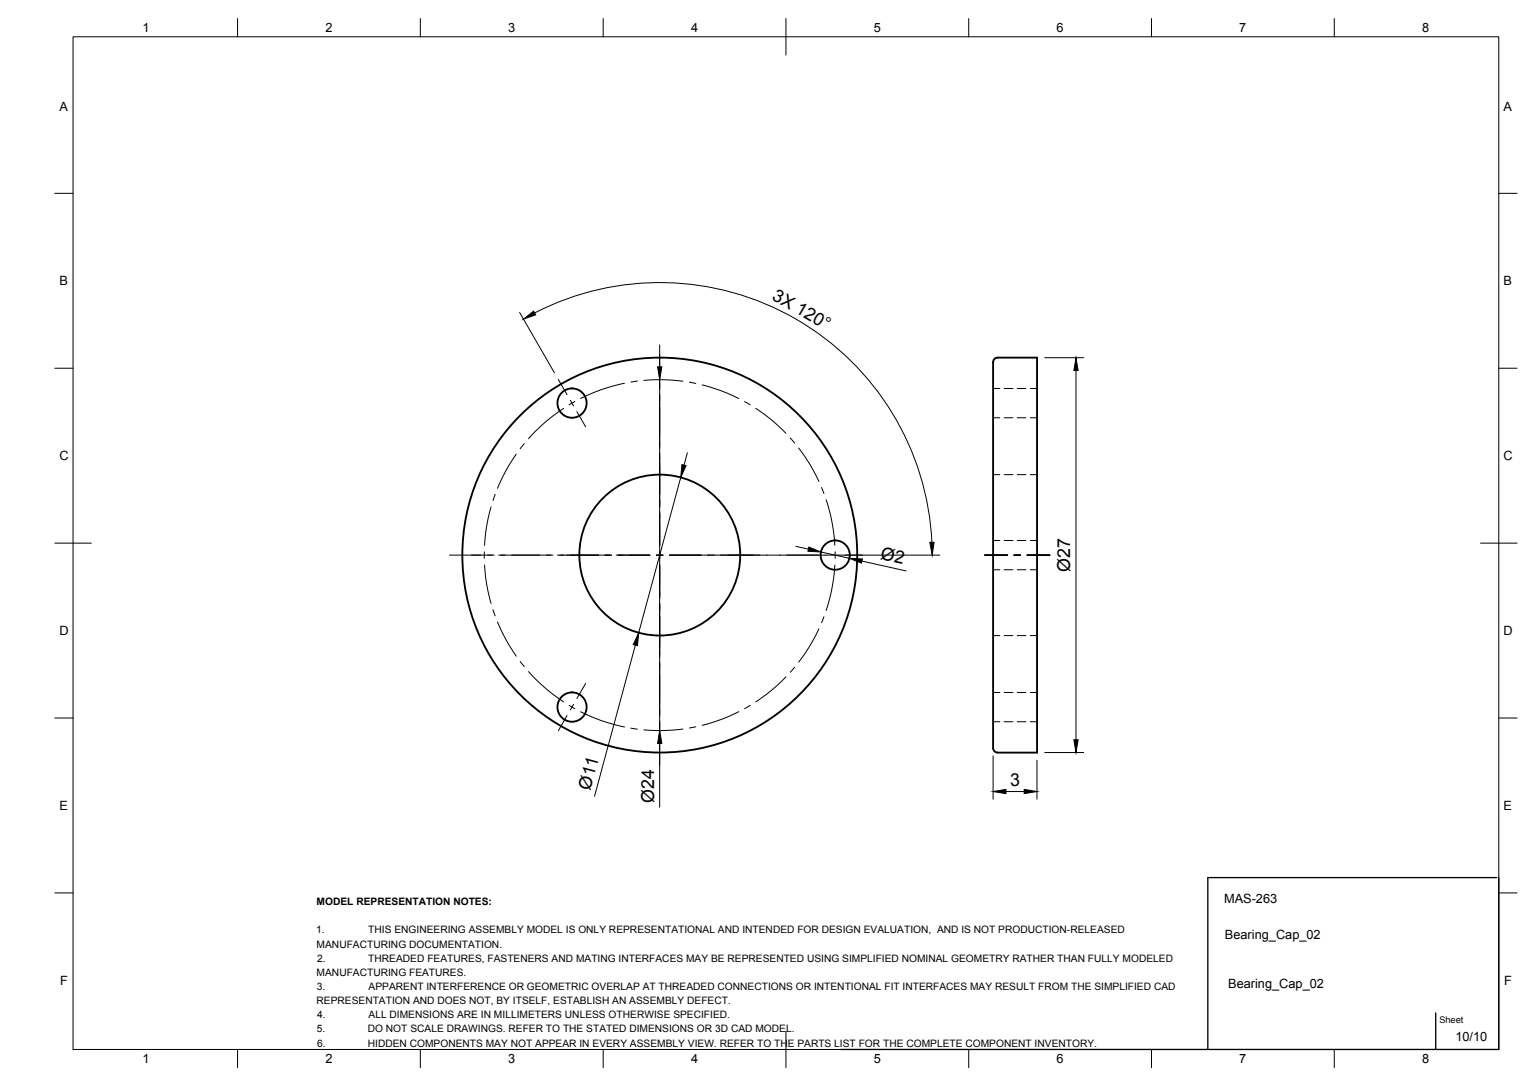
ISO-10303-21;
HEADER;
/* Generated by software containing ST-Developer
 * from STEP Tools, Inc. (www.steptools.com) 
 */

FILE_DESCRIPTION(
/* description */ (''),
/* implementation_level */ '2;1');

FILE_NAME(
/* name */ 'Bearing_Cap_02.step',
/* time_stamp */ '2026-10-12T15:47:30-07:00',
/* author */ (''),
/* organization */ (''),
/* preprocessor_version */ 'ST-DEVELOPER v20.2',
/* originating_system */ 'Autodesk Translation Framework v15.15.0.0',
/* authorisation */ '');

FILE_SCHEMA (('AUTOMOTIVE_DESIGN { 1 0 10303 214 3 1 1 }'));
ENDSEC;

DATA;
#10=MECHANICAL_DESIGN_GEOMETRIC_PRESENTATION_REPRESENTATION('',(#88),#88483);
#70=SHAPE_REPRESENTATION_RELATIONSHIP('SRR','None',#88526,#79);
#79=ADVANCED_BREP_SHAPE_REPRESENTATION('',(#123),#88480);
#88=STYLED_ITEM('',(#88574),#123);
#123=MANIFOLD_SOLID_BREP('Body1',#12998);
#174=TOROIDAL_SURFACE('',#13981,13.2,0.3);
#399=FACE_BOUND('',#2026,.T.);
#400=FACE_BOUND('',#2027,.T.);
#401=FACE_BOUND('',#2028,.T.);
#402=FACE_BOUND('',#2029,.T.);
#403=FACE_BOUND('',#2032,.T.);
#404=FACE_BOUND('',#2033,.T.);
#405=FACE_BOUND('',#2034,.T.);
#406=FACE_BOUND('',#2035,.T.);
#551=PLANE('',#13988);
#552=PLANE('',#13992);
#1302=FACE_OUTER_BOUND('',#2020,.T.);
#1303=FACE_OUTER_BOUND('',#2021,.T.);
#1304=FACE_OUTER_BOUND('',#2022,.T.);
#1305=FACE_OUTER_BOUND('',#2023,.T.);
#1306=FACE_OUTER_BOUND('',#2024,.T.);
#1307=FACE_OUTER_BOUND('',#2025,.T.);
#1308=FACE_OUTER_BOUND('',#2030,.T.);
#1309=FACE_OUTER_BOUND('',#2031,.T.);
#2020=EDGE_LOOP('',(#11452,#11453,#11454,#11455));
#2021=EDGE_LOOP('',(#11456,#11457,#11458,#11459));
#2022=EDGE_LOOP('',(#11460,#11461,#11462,#11463));
#2023=EDGE_LOOP('',(#11464,#11465,#11466,#11467,#11468));
#2024=EDGE_LOOP('',(#11469,#11470,#11471,#11472,#11473));
#2025=EDGE_LOOP('',(#11474));
#2026=EDGE_LOOP('',(#11475));
#2027=EDGE_LOOP('',(#11476));
#2028=EDGE_LOOP('',(#11477));
#2029=EDGE_LOOP('',(#11478));
#2030=EDGE_LOOP('',(#11479,#11480,#11481,#11482));
#2031=EDGE_LOOP('',(#11483));
#2032=EDGE_LOOP('',(#11484));
#2033=EDGE_LOOP('',(#11485));
#2034=EDGE_LOOP('',(#11486));
#2035=EDGE_LOOP('',(#11487));
#2686=CIRCLE('',#13973,1.);
#2687=CIRCLE('',#13974,1.);
#2688=CIRCLE('',#13976,1.);
#2689=CIRCLE('',#13977,1.);
#2690=CIRCLE('',#13979,1.);
#2691=CIRCLE('',#13980,1.);
#2692=CIRCLE('',#13982,13.2);
#2693=CIRCLE('',#13983,0.3);
#2694=CIRCLE('',#13984,13.5);
#2695=CIRCLE('',#13985,13.5);
#2696=CIRCLE('',#13987,13.5);
#2697=CIRCLE('',#13989,5.5);
#2698=CIRCLE('',#13991,5.5);
#4089=LINE('',#87468,#4559);
#4090=LINE('',#87474,#4560);
#4091=LINE('',#87480,#4561);
#4092=LINE('',#87493,#4562);
#4093=LINE('',#87499,#4563);
#4559=VECTOR('',#16487,1.);
#4560=VECTOR('',#16494,1.);
#4561=VECTOR('',#16501,1.);
#4562=VECTOR('',#16518,13.5);
#4563=VECTOR('',#16525,5.5);
#5821=VERTEX_POINT('',#87465);
#5822=VERTEX_POINT('',#87467);
#5823=VERTEX_POINT('',#87471);
#5824=VERTEX_POINT('',#87473);
#5825=VERTEX_POINT('',#87477);
#5826=VERTEX_POINT('',#87479);
#5827=VERTEX_POINT('',#87483);
#5828=VERTEX_POINT('',#87485);
#5829=VERTEX_POINT('',#87487);
#5830=VERTEX_POINT('',#87491);
#5831=VERTEX_POINT('',#87495);
#5832=VERTEX_POINT('',#87498);
#7738=EDGE_CURVE('',#5821,#5821,#2686,.T.);
#7739=EDGE_CURVE('',#5821,#5822,#4089,.T.);
#7740=EDGE_CURVE('',#5822,#5822,#2687,.T.);
#7741=EDGE_CURVE('',#5823,#5823,#2688,.T.);
#7742=EDGE_CURVE('',#5823,#5824,#4090,.T.);
#7743=EDGE_CURVE('',#5824,#5824,#2689,.T.);
#7744=EDGE_CURVE('',#5825,#5825,#2690,.T.);
#7745=EDGE_CURVE('',#5825,#5826,#4091,.T.);
#7746=EDGE_CURVE('',#5826,#5826,#2691,.T.);
#7747=EDGE_CURVE('',#5827,#5827,#2692,.T.);
#7748=EDGE_CURVE('',#5827,#5828,#2693,.T.);
#7749=EDGE_CURVE('',#5829,#5828,#2694,.T.);
#7750=EDGE_CURVE('',#5828,#5829,#2695,.T.);
#7751=EDGE_CURVE('',#5830,#5830,#2696,.T.);
#7752=EDGE_CURVE('',#5830,#5829,#4092,.T.);
#7753=EDGE_CURVE('',#5831,#5831,#2697,.T.);
#7754=EDGE_CURVE('',#5831,#5832,#4093,.T.);
#7755=EDGE_CURVE('',#5832,#5832,#2698,.T.);
#11452=ORIENTED_EDGE('',*,*,#7738,.T.);
#11453=ORIENTED_EDGE('',*,*,#7739,.T.);
#11454=ORIENTED_EDGE('',*,*,#7740,.T.);
#11455=ORIENTED_EDGE('',*,*,#7739,.F.);
#11456=ORIENTED_EDGE('',*,*,#7741,.T.);
#11457=ORIENTED_EDGE('',*,*,#7742,.T.);
#11458=ORIENTED_EDGE('',*,*,#7743,.T.);
#11459=ORIENTED_EDGE('',*,*,#7742,.F.);
#11460=ORIENTED_EDGE('',*,*,#7744,.T.);
#11461=ORIENTED_EDGE('',*,*,#7745,.T.);
#11462=ORIENTED_EDGE('',*,*,#7746,.T.);
#11463=ORIENTED_EDGE('',*,*,#7745,.F.);
#11464=ORIENTED_EDGE('',*,*,#7747,.F.);
#11465=ORIENTED_EDGE('',*,*,#7748,.T.);
#11466=ORIENTED_EDGE('',*,*,#7749,.F.);
#11467=ORIENTED_EDGE('',*,*,#7750,.F.);
#11468=ORIENTED_EDGE('',*,*,#7748,.F.);
#11469=ORIENTED_EDGE('',*,*,#7751,.F.);
#11470=ORIENTED_EDGE('',*,*,#7752,.T.);
#11471=ORIENTED_EDGE('',*,*,#7749,.T.);
#11472=ORIENTED_EDGE('',*,*,#7750,.T.);
#11473=ORIENTED_EDGE('',*,*,#7752,.F.);
#11474=ORIENTED_EDGE('',*,*,#7747,.T.);
#11475=ORIENTED_EDGE('',*,*,#7740,.F.);
#11476=ORIENTED_EDGE('',*,*,#7743,.F.);
#11477=ORIENTED_EDGE('',*,*,#7746,.F.);
#11478=ORIENTED_EDGE('',*,*,#7753,.F.);
#11479=ORIENTED_EDGE('',*,*,#7753,.T.);
#11480=ORIENTED_EDGE('',*,*,#7754,.T.);
#11481=ORIENTED_EDGE('',*,*,#7755,.F.);
#11482=ORIENTED_EDGE('',*,*,#7754,.F.);
#11483=ORIENTED_EDGE('',*,*,#7751,.T.);
#11484=ORIENTED_EDGE('',*,*,#7738,.F.);
#11485=ORIENTED_EDGE('',*,*,#7741,.F.);
#11486=ORIENTED_EDGE('',*,*,#7744,.F.);
#11487=ORIENTED_EDGE('',*,*,#7755,.T.);
#12271=CYLINDRICAL_SURFACE('',#13972,1.);
#12272=CYLINDRICAL_SURFACE('',#13975,1.);
#12273=CYLINDRICAL_SURFACE('',#13978,1.);
#12274=CYLINDRICAL_SURFACE('',#13986,13.5);
#12275=CYLINDRICAL_SURFACE('',#13990,5.5);
#12832=ADVANCED_FACE('',(#1302),#12271,.F.);
#12833=ADVANCED_FACE('',(#1303),#12272,.F.);
#12834=ADVANCED_FACE('',(#1304),#12273,.F.);
#12835=ADVANCED_FACE('',(#1305),#174,.T.);
#12836=ADVANCED_FACE('',(#1306),#12274,.T.);
#12837=ADVANCED_FACE('',(#1307,#399,#400,#401,#402),#551,.F.);
#12838=ADVANCED_FACE('',(#1308),#12275,.F.);
#12839=ADVANCED_FACE('',(#1309,#403,#404,#405,#406),#552,.T.);
#12998=CLOSED_SHELL('',(#12832,#12833,#12834,#12835,#12836,#12837,#12838,
#12839));
#13971=AXIS2_PLACEMENT_3D('',#87463,#16481,#16482);
#13972=AXIS2_PLACEMENT_3D('',#87464,#16483,#16484);
#13973=AXIS2_PLACEMENT_3D('',#87466,#16485,#16486);
#13974=AXIS2_PLACEMENT_3D('',#87469,#16488,#16489);
#13975=AXIS2_PLACEMENT_3D('',#87470,#16490,#16491);
#13976=AXIS2_PLACEMENT_3D('',#87472,#16492,#16493);
#13977=AXIS2_PLACEMENT_3D('',#87475,#16495,#16496);
#13978=AXIS2_PLACEMENT_3D('',#87476,#16497,#16498);
#13979=AXIS2_PLACEMENT_3D('',#87478,#16499,#16500);
#13980=AXIS2_PLACEMENT_3D('',#87481,#16502,#16503);
#13981=AXIS2_PLACEMENT_3D('',#87482,#16504,#16505);
#13982=AXIS2_PLACEMENT_3D('',#87484,#16506,#16507);
#13983=AXIS2_PLACEMENT_3D('',#87486,#16508,#16509);
#13984=AXIS2_PLACEMENT_3D('',#87488,#16510,#16511);
#13985=AXIS2_PLACEMENT_3D('',#87489,#16512,#16513);
#13986=AXIS2_PLACEMENT_3D('',#87490,#16514,#16515);
#13987=AXIS2_PLACEMENT_3D('',#87492,#16516,#16517);
#13988=AXIS2_PLACEMENT_3D('',#87494,#16519,#16520);
#13989=AXIS2_PLACEMENT_3D('',#87496,#16521,#16522);
#13990=AXIS2_PLACEMENT_3D('',#87497,#16523,#16524);
#13991=AXIS2_PLACEMENT_3D('',#87500,#16526,#16527);
#13992=AXIS2_PLACEMENT_3D('',#87501,#16528,#16529);
#16481=DIRECTION('axis',(0.,0.,1.));
#16482=DIRECTION('refdir',(1.,0.,0.));
#16483=DIRECTION('center_axis',(-1.,0.,0.));
#16484=DIRECTION('ref_axis',(0.,1.,0.));
#16485=DIRECTION('center_axis',(1.,0.,0.));
#16486=DIRECTION('ref_axis',(0.,1.,0.));
#16487=DIRECTION('',(-1.,0.,0.));
#16488=DIRECTION('center_axis',(-1.,0.,0.));
#16489=DIRECTION('ref_axis',(0.,1.,0.));
#16490=DIRECTION('center_axis',(-1.,0.,0.));
#16491=DIRECTION('ref_axis',(0.,1.,0.));
#16492=DIRECTION('center_axis',(1.,0.,0.));
#16493=DIRECTION('ref_axis',(0.,1.,0.));
#16494=DIRECTION('',(-1.,0.,0.));
#16495=DIRECTION('center_axis',(-1.,0.,0.));
#16496=DIRECTION('ref_axis',(0.,1.,0.));
#16497=DIRECTION('center_axis',(-1.,0.,0.));
#16498=DIRECTION('ref_axis',(0.,1.,0.));
#16499=DIRECTION('center_axis',(1.,0.,0.));
#16500=DIRECTION('ref_axis',(0.,1.,0.));
#16501=DIRECTION('',(-1.,0.,0.));
#16502=DIRECTION('center_axis',(-1.,0.,0.));
#16503=DIRECTION('ref_axis',(0.,1.,0.));
#16504=DIRECTION('center_axis',(-1.,0.,0.));
#16505=DIRECTION('ref_axis',(0.,0.,-1.));
#16506=DIRECTION('center_axis',(-1.,0.,0.));
#16507=DIRECTION('ref_axis',(0.,0.342020143325669,0.939692620785908));
#16508=DIRECTION('center_axis',(0.,1.,0.));
#16509=DIRECTION('ref_axis',(0.,0.,1.));
#16510=DIRECTION('center_axis',(1.,0.,0.));
#16511=DIRECTION('ref_axis',(0.,0.342020143325669,0.939692620785908));
#16512=DIRECTION('center_axis',(1.,0.,0.));
#16513=DIRECTION('ref_axis',(0.,0.342020143325669,0.939692620785908));
#16514=DIRECTION('center_axis',(1.,0.,0.));
#16515=DIRECTION('ref_axis',(0.,-0.296296296296299,-0.955096070979823));
#16516=DIRECTION('center_axis',(1.,0.,0.));
#16517=DIRECTION('ref_axis',(0.,-0.296296296296299,-0.955096070979823));
#16518=DIRECTION('',(-1.,0.,0.));
#16519=DIRECTION('center_axis',(1.,0.,0.));
#16520=DIRECTION('ref_axis',(0.,1.,0.));
#16521=DIRECTION('center_axis',(-1.,0.,0.));
#16522=DIRECTION('ref_axis',(0.,1.,0.));
#16523=DIRECTION('center_axis',(1.,0.,0.));
#16524=DIRECTION('ref_axis',(0.,1.,0.));
#16525=DIRECTION('',(1.,0.,0.));
#16526=DIRECTION('center_axis',(-1.,0.,0.));
#16527=DIRECTION('ref_axis',(0.,1.,0.));
#16528=DIRECTION('center_axis',(1.,0.,0.));
#16529=DIRECTION('ref_axis',(0.,1.,0.));
#87463=CARTESIAN_POINT('',(0.,0.,0.));
#87464=CARTESIAN_POINT('Origin',(-26.3408711739,15.6090782051017,5.99920149541289));
#87465=CARTESIAN_POINT('',(-23.3408711739,14.6090782051017,5.99920149541289));
#87466=CARTESIAN_POINT('Origin',(-23.3408711739,15.6090782051017,5.99920149541289));
#87467=CARTESIAN_POINT('',(-26.3408711739,14.6090782051017,5.99920149541289));
#87468=CARTESIAN_POINT('',(-26.3408711739,14.6090782051017,5.99920149541289));
#87469=CARTESIAN_POINT('Origin',(-26.3408711739,15.6090782051017,5.99920149541289));
#87470=CARTESIAN_POINT('Origin',(-26.3408711739,36.3909217948983,5.99920149541289));
#87471=CARTESIAN_POINT('',(-23.3408711739,35.3909217948983,5.99920149541289));
#87472=CARTESIAN_POINT('Origin',(-23.3408711739,36.3909217948983,5.99920149541289));
#87473=CARTESIAN_POINT('',(-26.3408711739,35.3909217948983,5.99920149541289));
#87474=CARTESIAN_POINT('',(-26.3408711739,35.3909217948983,5.99920149541289));
#87475=CARTESIAN_POINT('Origin',(-26.3408711739,36.3909217948983,5.99920149541289));
#87476=CARTESIAN_POINT('Origin',(-26.3408711739,26.,-11.9984029908258));
#87477=CARTESIAN_POINT('',(-23.3408711739,25.,-11.9984029908258));
#87478=CARTESIAN_POINT('Origin',(-23.3408711739,26.,-11.9984029908258));
#87479=CARTESIAN_POINT('',(-26.3408711739,25.,-11.9984029908258));
#87480=CARTESIAN_POINT('',(-26.3408711739,25.,-11.9984029908258));
#87481=CARTESIAN_POINT('Origin',(-26.3408711739,26.,-11.9984029908258));
#87482=CARTESIAN_POINT('Origin',(-26.0408711739,26.,7.77156117237612E-15));
#87483=CARTESIAN_POINT('',(-26.3408711739,26.,13.2));
#87484=CARTESIAN_POINT('Origin',(-26.3408711739,26.,7.77156117237612E-15));
#87485=CARTESIAN_POINT('',(-26.0408711739,26.,13.5));
#87486=CARTESIAN_POINT('Origin',(-26.0408711739,26.,13.2));
#87487=CARTESIAN_POINT('',(-26.0408711739,30.,12.8937969582276));
#87488=CARTESIAN_POINT('Origin',(-26.0408711739,26.,7.77156117237612E-15));
#87489=CARTESIAN_POINT('Origin',(-26.0408711739,26.,7.77156117237612E-15));
#87490=CARTESIAN_POINT('Origin',(-23.3408711739,26.,7.77156117237612E-15));
#87491=CARTESIAN_POINT('',(-23.3408711739,30.,12.8937969582276));
#87492=CARTESIAN_POINT('Origin',(-23.3408711739,26.,7.77156117237612E-15));
#87493=CARTESIAN_POINT('',(-23.3408711739,30.,12.8937969582276));
#87494=CARTESIAN_POINT('Origin',(-26.3408711739,26.,1.11022302462516E-14));
#87495=CARTESIAN_POINT('',(-26.3408711739,20.5,7.09800543284508E-15));
#87496=CARTESIAN_POINT('Origin',(-26.3408711739,26.,7.77156117237612E-15));
#87497=CARTESIAN_POINT('Origin',(-23.3408711739,26.,7.77156117237612E-15));
#87498=CARTESIAN_POINT('',(-23.3408711739,20.5,7.09800543284508E-15));
#87499=CARTESIAN_POINT('',(-23.3408711739,20.5,7.09800543284507E-15));
#87500=CARTESIAN_POINT('Origin',(-23.3408711739,26.,7.77156117237612E-15));
#87501=CARTESIAN_POINT('Origin',(-23.3408711739,26.,1.11022302462516E-14));
#88469=UNCERTAINTY_MEASURE_WITH_UNIT(LENGTH_MEASURE(0.01),#88484,
'DISTANCE_ACCURACY_VALUE',
'Maximum model space distance between geometric entities at asserted c
onnectivities');
#88472=UNCERTAINTY_MEASURE_WITH_UNIT(LENGTH_MEASURE(0.01),#88484,
'DISTANCE_ACCURACY_VALUE',
'Maximum model space distance between geometric entities at asserted c
onnectivities');
#88480=(
GEOMETRIC_REPRESENTATION_CONTEXT(3)
GLOBAL_UNCERTAINTY_ASSIGNED_CONTEXT((#88469))
GLOBAL_UNIT_ASSIGNED_CONTEXT((#88484,#88486,#88487))
REPRESENTATION_CONTEXT('','3D')
);
#88483=(
GEOMETRIC_REPRESENTATION_CONTEXT(3)
GLOBAL_UNCERTAINTY_ASSIGNED_CONTEXT((#88472))
GLOBAL_UNIT_ASSIGNED_CONTEXT((#88484,#88486,#88487))
REPRESENTATION_CONTEXT('','3D')
);
#88484=(
LENGTH_UNIT()
NAMED_UNIT(*)
SI_UNIT(.MILLI.,.METRE.)
);
#88486=(
NAMED_UNIT(*)
PLANE_ANGLE_UNIT()
SI_UNIT($,.RADIAN.)
);
#88487=(
NAMED_UNIT(*)
SI_UNIT($,.STERADIAN.)
SOLID_ANGLE_UNIT()
);
#88495=SHAPE_DEFINITION_REPRESENTATION(#88505,#88526);
#88505=PRODUCT_DEFINITION_SHAPE('',$,#88537);
#88526=SHAPE_REPRESENTATION('',(#13971),#88480);
#88529=PRODUCT_DEFINITION_CONTEXT('part definition',#88561,'design');
#88537=PRODUCT_DEFINITION('Bearing_Cap_02','Bearing_Cap_02',#88547,#88529);
#88547=PRODUCT_DEFINITION_FORMATION('',$,#88570);
#88561=APPLICATION_CONTEXT(
'Core Data for Automotive Mechanical Design Process');
#88562=PRODUCT_CONTEXT('part definition',#88561,'mechanical');
#88570=PRODUCT('Bearing_Cap_02','Bearing_Cap_02',$,(#88562));
#88574=PRESENTATION_STYLE_ASSIGNMENT((#88576));
#88576=SURFACE_STYLE_USAGE(.BOTH.,#88578);
#88578=SURFACE_SIDE_STYLE('',(#88580));
#88580=SURFACE_STYLE_FILL_AREA(#88582);
#88582=FILL_AREA_STYLE('Opaque(160,160,160)',(#88584));
#88584=FILL_AREA_STYLE_COLOUR('Opaque(160,160,160)',#88586);
#88586=COLOUR_RGB('Opaque(160,160,160)', 0.66274510, 0.83137255, 0.94901961);
ENDSEC;
END-ISO-10303-21;
